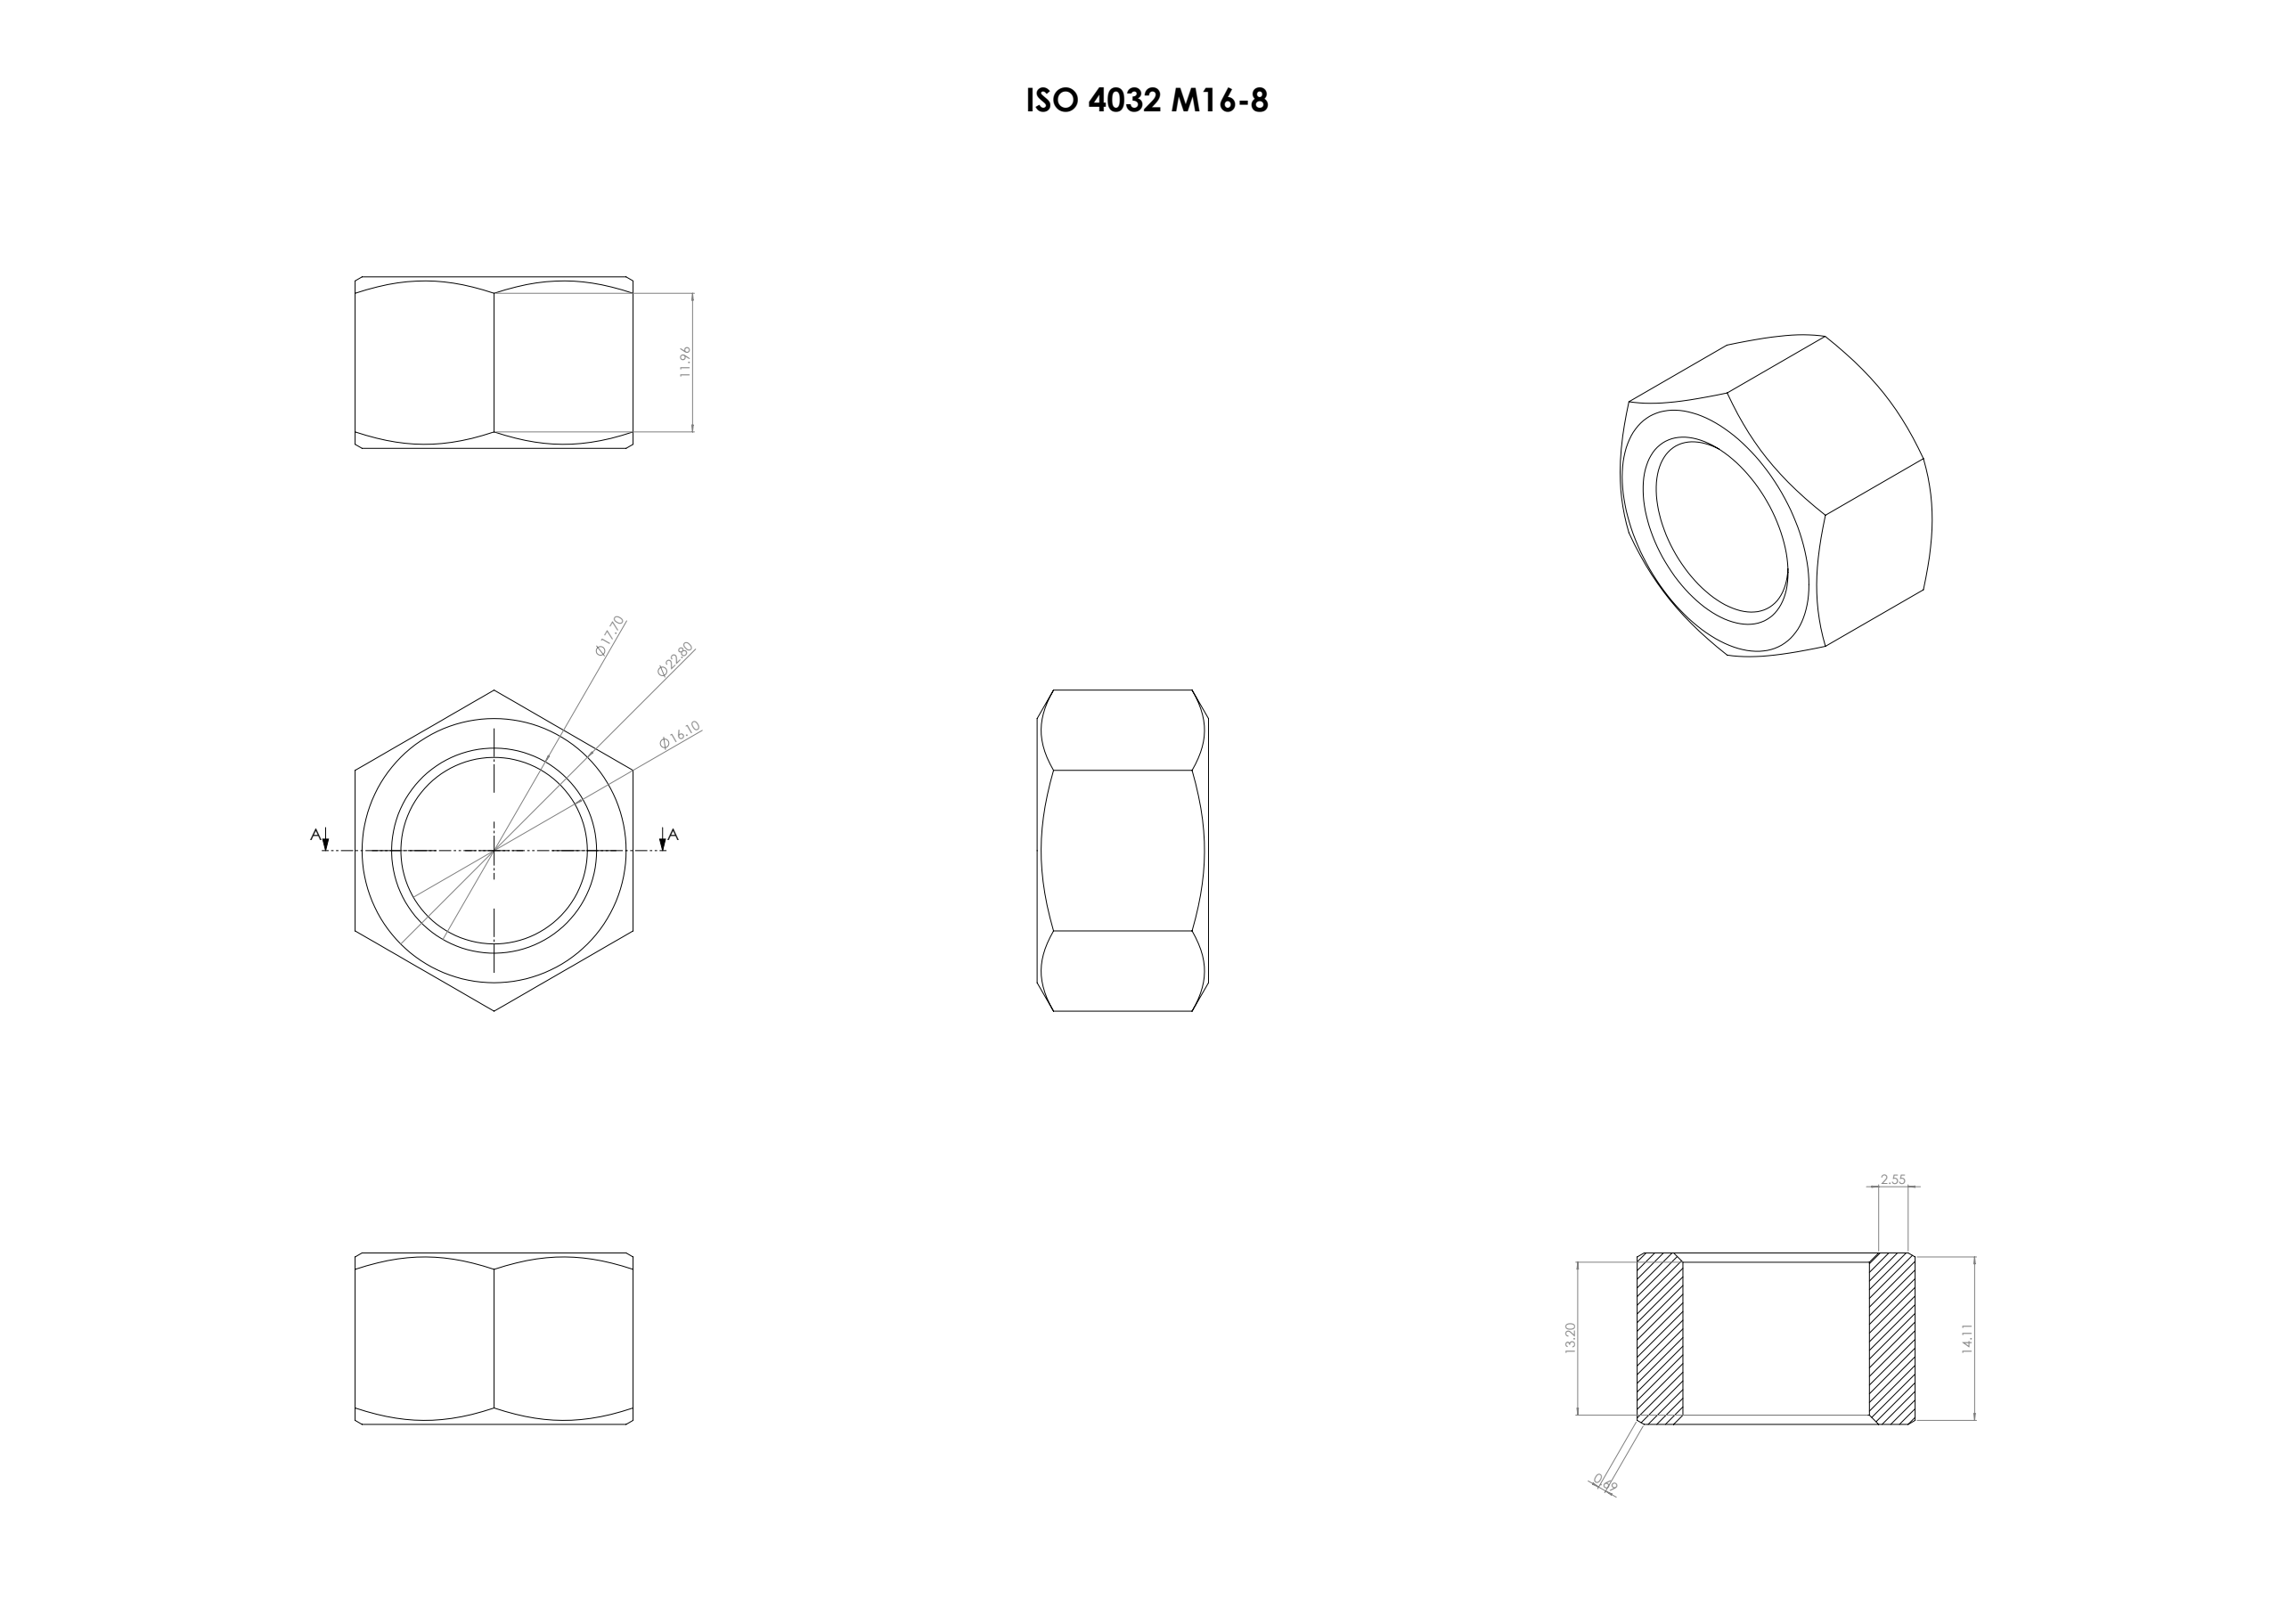
ISO-10303-21;
HEADER;
/* Generated by software containing ST-Developer
 * from STEP Tools, Inc. (www.steptools.com) 
 */

FILE_DESCRIPTION(
/* description */ (''),
/* implementation_level */ '2;1');

FILE_NAME(
/* name */ '18_ISO_4032_M16-8.step',
/* time_stamp */ '2026-10-20T10:03:03-07:00',
/* author */ (''),
/* organization */ (''),
/* preprocessor_version */ 'ST-DEVELOPER v20.2',
/* originating_system */ 'Autodesk Translation Framework v15.15.0.0',
/* authorisation */ '');

FILE_SCHEMA (('AUTOMOTIVE_DESIGN { 1 0 10303 214 3 1 1 }'));
ENDSEC;

DATA;
#10=MECHANICAL_DESIGN_GEOMETRIC_PRESENTATION_REPRESENTATION('',(#540),#71492);
#362=(
BOUNDED_CURVE()
B_SPLINE_CURVE(2,(#70596,#70597,#70598),.UNSPECIFIED.,.F.,.F.)
B_SPLINE_CURVE_WITH_KNOTS((3,3),(0.083069206448341,0.799733019594622),
 .UNSPECIFIED.)
CURVE()
GEOMETRIC_REPRESENTATION_ITEM()
RATIONAL_B_SPLINE_CURVE((1.01933756729741,1.09818360252296,1.09818360252296))
REPRESENTATION_ITEM('')
);
#363=(
BOUNDED_CURVE()
B_SPLINE_CURVE(2,(#70600,#70601,#70602),.UNSPECIFIED.,.F.,.F.)
B_SPLINE_CURVE_WITH_KNOTS((3,3),(0.0830692064483412,1.5163968327409),
 .UNSPECIFIED.)
CURVE()
GEOMETRIC_REPRESENTATION_ITEM()
RATIONAL_B_SPLINE_CURVE((1.01933756729741,1.17702963774851,1.01933756729741))
REPRESENTATION_ITEM('')
);
#364=(
BOUNDED_CURVE()
B_SPLINE_CURVE(2,(#70604,#70605,#70606),.UNSPECIFIED.,.F.,.F.)
B_SPLINE_CURVE_WITH_KNOTS((3,3),(0.0830692064483411,1.5163968327409),
 .UNSPECIFIED.)
CURVE()
GEOMETRIC_REPRESENTATION_ITEM()
RATIONAL_B_SPLINE_CURVE((1.01933756729741,1.17702963774851,1.01933756729741))
REPRESENTATION_ITEM('')
);
#365=(
BOUNDED_CURVE()
B_SPLINE_CURVE(2,(#70608,#70609,#70610),.UNSPECIFIED.,.F.,.F.)
B_SPLINE_CURVE_WITH_KNOTS((3,3),(0.0830692064483411,1.5163968327409),
 .UNSPECIFIED.)
CURVE()
GEOMETRIC_REPRESENTATION_ITEM()
RATIONAL_B_SPLINE_CURVE((1.01933756729741,1.17702963774851,1.01933756729741))
REPRESENTATION_ITEM('')
);
#366=(
BOUNDED_CURVE()
B_SPLINE_CURVE(2,(#70612,#70613,#70614),.UNSPECIFIED.,.F.,.F.)
B_SPLINE_CURVE_WITH_KNOTS((3,3),(0.083069206448341,1.5163968327409),
 .UNSPECIFIED.)
CURVE()
GEOMETRIC_REPRESENTATION_ITEM()
RATIONAL_B_SPLINE_CURVE((1.01933756729741,1.17702963774852,1.01933756729741))
REPRESENTATION_ITEM('')
);
#367=(
BOUNDED_CURVE()
B_SPLINE_CURVE(2,(#70616,#70617,#70618),.UNSPECIFIED.,.F.,.F.)
B_SPLINE_CURVE_WITH_KNOTS((3,3),(0.0830692064483414,1.5163968327409),
 .UNSPECIFIED.)
CURVE()
GEOMETRIC_REPRESENTATION_ITEM()
RATIONAL_B_SPLINE_CURVE((1.01933756729741,1.17702963774851,1.01933756729741))
REPRESENTATION_ITEM('')
);
#368=(
BOUNDED_CURVE()
B_SPLINE_CURVE(2,(#70619,#70620,#70621),.UNSPECIFIED.,.F.,.F.)
B_SPLINE_CURVE_WITH_KNOTS((3,3),(0.799733019594622,1.5163968327409),
 .UNSPECIFIED.)
CURVE()
GEOMETRIC_REPRESENTATION_ITEM()
RATIONAL_B_SPLINE_CURVE((1.09818360252296,1.09818360252296,1.01933756729741))
REPRESENTATION_ITEM('')
);
#369=(
BOUNDED_CURVE()
B_SPLINE_CURVE(2,(#70626,#70627,#70628),.UNSPECIFIED.,.F.,.F.)
B_SPLINE_CURVE_WITH_KNOTS((3,3),(0.0830692064483413,1.5163968327409),
 .UNSPECIFIED.)
CURVE()
GEOMETRIC_REPRESENTATION_ITEM()
RATIONAL_B_SPLINE_CURVE((1.01933756729741,1.17702963774851,1.01933756729741))
REPRESENTATION_ITEM('')
);
#370=(
BOUNDED_CURVE()
B_SPLINE_CURVE(2,(#70633,#70634,#70635),.UNSPECIFIED.,.F.,.F.)
B_SPLINE_CURVE_WITH_KNOTS((3,3),(0.0830692064483417,1.5163968327409),
 .UNSPECIFIED.)
CURVE()
GEOMETRIC_REPRESENTATION_ITEM()
RATIONAL_B_SPLINE_CURVE((1.01933756729741,1.17702963774851,1.01933756729741))
REPRESENTATION_ITEM('')
);
#371=(
BOUNDED_CURVE()
B_SPLINE_CURVE(2,(#70639,#70640,#70641),.UNSPECIFIED.,.F.,.F.)
B_SPLINE_CURVE_WITH_KNOTS((3,3),(0.0830692064483414,1.5163968327409),
 .UNSPECIFIED.)
CURVE()
GEOMETRIC_REPRESENTATION_ITEM()
RATIONAL_B_SPLINE_CURVE((1.01933756729741,1.17702963774851,1.01933756729741))
REPRESENTATION_ITEM('')
);
#372=(
BOUNDED_CURVE()
B_SPLINE_CURVE(2,(#70644,#70645,#70646),.UNSPECIFIED.,.F.,.F.)
B_SPLINE_CURVE_WITH_KNOTS((3,3),(0.0830692064483411,1.5163968327409),
 .UNSPECIFIED.)
CURVE()
GEOMETRIC_REPRESENTATION_ITEM()
RATIONAL_B_SPLINE_CURVE((1.01933756729741,1.17702963774851,1.01933756729741))
REPRESENTATION_ITEM('')
);
#373=(
BOUNDED_CURVE()
B_SPLINE_CURVE(2,(#70648,#70649,#70650),.UNSPECIFIED.,.F.,.F.)
B_SPLINE_CURVE_WITH_KNOTS((3,3),(0.799733019594622,1.5163968327409),
 .UNSPECIFIED.)
CURVE()
GEOMETRIC_REPRESENTATION_ITEM()
RATIONAL_B_SPLINE_CURVE((1.09818360252296,1.09818360252296,1.01933756729741))
REPRESENTATION_ITEM('')
);
#374=(
BOUNDED_CURVE()
B_SPLINE_CURVE(2,(#70653,#70654,#70655),.UNSPECIFIED.,.F.,.F.)
B_SPLINE_CURVE_WITH_KNOTS((3,3),(0.0830692064483414,0.799733019594622),
 .UNSPECIFIED.)
CURVE()
GEOMETRIC_REPRESENTATION_ITEM()
RATIONAL_B_SPLINE_CURVE((1.01933756729741,1.09818360252296,1.09818360252296))
REPRESENTATION_ITEM('')
);
#375=(
BOUNDED_CURVE()
B_SPLINE_CURVE(2,(#70656,#70657,#70658),.UNSPECIFIED.,.F.,.F.)
B_SPLINE_CURVE_WITH_KNOTS((3,3),(0.0830692064483413,1.5163968327409),
 .UNSPECIFIED.)
CURVE()
GEOMETRIC_REPRESENTATION_ITEM()
RATIONAL_B_SPLINE_CURVE((1.01933756729741,1.17702963774851,1.01933756729741))
REPRESENTATION_ITEM('')
);
#397=SHAPE_REPRESENTATION_RELATIONSHIP('SRR','None',#71618,#416);
#416=ADVANCED_BREP_SHAPE_REPRESENTATION('',(#435),#71488);
#435=MANIFOLD_SOLID_BREP('Nut',#28474);
#540=STYLED_ITEM('',(#71894),#435);
#1830=CYLINDRICAL_SURFACE('',#30448,0.805);
#1984=FACE_BOUND('',#6070,.T.);
#1985=FACE_BOUND('',#6073,.T.);
#2563=CIRCLE('',#30446,0.805);
#2564=CIRCLE('',#30447,0.885);
#2565=CIRCLE('',#30449,0.805);
#2566=CIRCLE('',#30451,1.14);
#2567=CIRCLE('',#30453,0.885);
#2568=CIRCLE('',#30455,1.14);
#2895=CONICAL_SURFACE('',#30445,0.845,0.785398163397448);
#2896=CONICAL_SURFACE('',#30452,0.845,0.785398163397448);
#2897=CONICAL_SURFACE('',#30456,1.28782032302755,1.0471975511966);
#2898=CONICAL_SURFACE('',#30460,1.28782032302755,1.0471975511966);
#4377=FACE_OUTER_BOUND('',#6067,.T.);
#4378=FACE_OUTER_BOUND('',#6068,.T.);
#4379=FACE_OUTER_BOUND('',#6069,.T.);
#4380=FACE_OUTER_BOUND('',#6071,.T.);
#4381=FACE_OUTER_BOUND('',#6072,.T.);
#4382=FACE_OUTER_BOUND('',#6074,.T.);
#4383=FACE_OUTER_BOUND('',#6075,.T.);
#4384=FACE_OUTER_BOUND('',#6076,.T.);
#4385=FACE_OUTER_BOUND('',#6077,.T.);
#4386=FACE_OUTER_BOUND('',#6078,.T.);
#4387=FACE_OUTER_BOUND('',#6079,.T.);
#4388=FACE_OUTER_BOUND('',#6080,.T.);
#4389=FACE_OUTER_BOUND('',#6081,.T.);
#6067=EDGE_LOOP('',(#25305,#25306,#25307,#25308));
#6068=EDGE_LOOP('',(#25309,#25310,#25311,#25312));
#6069=EDGE_LOOP('',(#25313));
#6070=EDGE_LOOP('',(#25314));
#6071=EDGE_LOOP('',(#25315,#25316,#25317,#25318));
#6072=EDGE_LOOP('',(#25319));
#6073=EDGE_LOOP('',(#25320));
#6074=EDGE_LOOP('',(#25321,#25322,#25323,#25324,#25325,#25326,#25327,#25328,
#25329,#25330));
#6075=EDGE_LOOP('',(#25331,#25332,#25333,#25334));
#6076=EDGE_LOOP('',(#25335,#25336,#25337,#25338));
#6077=EDGE_LOOP('',(#25339,#25340,#25341,#25342));
#6078=EDGE_LOOP('',(#25343,#25344,#25345,#25346,#25347,#25348,#25349,#25350,
#25351,#25352));
#6079=EDGE_LOOP('',(#25353,#25354,#25355,#25356));
#6080=EDGE_LOOP('',(#25357,#25358,#25359,#25360));
#6081=EDGE_LOOP('',(#25361,#25362,#25363,#25364,#25365,#25366));
#8589=LINE('',#70576,#11077);
#8590=LINE('',#70581,#11078);
#8591=LINE('',#70588,#11079);
#8592=LINE('',#70594,#11080);
#8593=LINE('',#70624,#11081);
#8594=LINE('',#70629,#11082);
#8595=LINE('',#70632,#11083);
#8596=LINE('',#70638,#11084);
#8597=LINE('',#70651,#11085);
#8598=LINE('',#70660,#11086);
#8599=LINE('',#70662,#11087);
#11077=VECTOR('',#36660,0.845);
#11078=VECTOR('',#36667,0.805);
#11079=VECTOR('',#36676,0.845);
#11080=VECTOR('',#36683,1.28782032302755);
#11081=VECTOR('',#36686,1.);
#11082=VECTOR('',#36687,1.);
#11083=VECTOR('',#36690,1.);
#11084=VECTOR('',#36693,1.);
#11085=VECTOR('',#36696,1.28782032302755);
#11086=VECTOR('',#36699,1.);
#11087=VECTOR('',#36702,1.);
#13617=VERTEX_POINT('',#70573);
#13618=VERTEX_POINT('',#70575);
#13619=VERTEX_POINT('',#70579);
#13620=VERTEX_POINT('',#70583);
#13621=VERTEX_POINT('',#70586);
#13622=VERTEX_POINT('',#70590);
#13623=VERTEX_POINT('',#70593);
#13624=VERTEX_POINT('',#70595);
#13625=VERTEX_POINT('',#70599);
#13626=VERTEX_POINT('',#70603);
#13627=VERTEX_POINT('',#70607);
#13628=VERTEX_POINT('',#70611);
#13629=VERTEX_POINT('',#70615);
#13630=VERTEX_POINT('',#70623);
#13631=VERTEX_POINT('',#70625);
#13632=VERTEX_POINT('',#70631);
#13633=VERTEX_POINT('',#70637);
#13634=VERTEX_POINT('',#70643);
#13635=VERTEX_POINT('',#70647);
#13636=VERTEX_POINT('',#70652);
#17536=EDGE_CURVE('',#13617,#13617,#2563,.T.);
#17537=EDGE_CURVE('',#13617,#13618,#8589,.T.);
#17538=EDGE_CURVE('',#13618,#13618,#2564,.T.);
#17539=EDGE_CURVE('',#13619,#13619,#2565,.T.);
#17540=EDGE_CURVE('',#13619,#13617,#8590,.T.);
#17541=EDGE_CURVE('',#13620,#13620,#2566,.T.);
#17542=EDGE_CURVE('',#13621,#13621,#2567,.T.);
#17543=EDGE_CURVE('',#13621,#13619,#8591,.T.);
#17544=EDGE_CURVE('',#13622,#13622,#2568,.T.);
#17545=EDGE_CURVE('',#13620,#13623,#8592,.T.);
#17546=EDGE_CURVE('',#13624,#13623,#362,.T.);
#17547=EDGE_CURVE('',#13625,#13624,#363,.T.);
#17548=EDGE_CURVE('',#13626,#13625,#364,.T.);
#17549=EDGE_CURVE('',#13627,#13626,#365,.T.);
#17550=EDGE_CURVE('',#13628,#13627,#366,.T.);
#17551=EDGE_CURVE('',#13629,#13628,#367,.T.);
#17552=EDGE_CURVE('',#13623,#13629,#368,.T.);
#17553=EDGE_CURVE('',#13627,#13630,#8593,.T.);
#17554=EDGE_CURVE('',#13630,#13631,#369,.T.);
#17555=EDGE_CURVE('',#13628,#13631,#8594,.T.);
#17556=EDGE_CURVE('',#13626,#13632,#8595,.T.);
#17557=EDGE_CURVE('',#13632,#13630,#370,.T.);
#17558=EDGE_CURVE('',#13625,#13633,#8596,.T.);
#17559=EDGE_CURVE('',#13633,#13632,#371,.T.);
#17560=EDGE_CURVE('',#13634,#13633,#372,.T.);
#17561=EDGE_CURVE('',#13635,#13634,#373,.T.);
#17562=EDGE_CURVE('',#13635,#13622,#8597,.T.);
#17563=EDGE_CURVE('',#13636,#13635,#374,.T.);
#17564=EDGE_CURVE('',#13631,#13636,#375,.T.);
#17565=EDGE_CURVE('',#13624,#13634,#8598,.T.);
#17566=EDGE_CURVE('',#13629,#13636,#8599,.T.);
#25305=ORIENTED_EDGE('',*,*,#17536,.T.);
#25306=ORIENTED_EDGE('',*,*,#17537,.T.);
#25307=ORIENTED_EDGE('',*,*,#17538,.T.);
#25308=ORIENTED_EDGE('',*,*,#17537,.F.);
#25309=ORIENTED_EDGE('',*,*,#17539,.F.);
#25310=ORIENTED_EDGE('',*,*,#17540,.T.);
#25311=ORIENTED_EDGE('',*,*,#17536,.F.);
#25312=ORIENTED_EDGE('',*,*,#17540,.F.);
#25313=ORIENTED_EDGE('',*,*,#17541,.T.);
#25314=ORIENTED_EDGE('',*,*,#17538,.F.);
#25315=ORIENTED_EDGE('',*,*,#17542,.T.);
#25316=ORIENTED_EDGE('',*,*,#17543,.T.);
#25317=ORIENTED_EDGE('',*,*,#17539,.T.);
#25318=ORIENTED_EDGE('',*,*,#17543,.F.);
#25319=ORIENTED_EDGE('',*,*,#17544,.T.);
#25320=ORIENTED_EDGE('',*,*,#17542,.F.);
#25321=ORIENTED_EDGE('',*,*,#17541,.F.);
#25322=ORIENTED_EDGE('',*,*,#17545,.T.);
#25323=ORIENTED_EDGE('',*,*,#17546,.F.);
#25324=ORIENTED_EDGE('',*,*,#17547,.F.);
#25325=ORIENTED_EDGE('',*,*,#17548,.F.);
#25326=ORIENTED_EDGE('',*,*,#17549,.F.);
#25327=ORIENTED_EDGE('',*,*,#17550,.F.);
#25328=ORIENTED_EDGE('',*,*,#17551,.F.);
#25329=ORIENTED_EDGE('',*,*,#17552,.F.);
#25330=ORIENTED_EDGE('',*,*,#17545,.F.);
#25331=ORIENTED_EDGE('',*,*,#17550,.T.);
#25332=ORIENTED_EDGE('',*,*,#17553,.T.);
#25333=ORIENTED_EDGE('',*,*,#17554,.T.);
#25334=ORIENTED_EDGE('',*,*,#17555,.F.);
#25335=ORIENTED_EDGE('',*,*,#17549,.T.);
#25336=ORIENTED_EDGE('',*,*,#17556,.T.);
#25337=ORIENTED_EDGE('',*,*,#17557,.T.);
#25338=ORIENTED_EDGE('',*,*,#17553,.F.);
#25339=ORIENTED_EDGE('',*,*,#17548,.T.);
#25340=ORIENTED_EDGE('',*,*,#17558,.T.);
#25341=ORIENTED_EDGE('',*,*,#17559,.T.);
#25342=ORIENTED_EDGE('',*,*,#17556,.F.);
#25343=ORIENTED_EDGE('',*,*,#17554,.F.);
#25344=ORIENTED_EDGE('',*,*,#17557,.F.);
#25345=ORIENTED_EDGE('',*,*,#17559,.F.);
#25346=ORIENTED_EDGE('',*,*,#17560,.F.);
#25347=ORIENTED_EDGE('',*,*,#17561,.F.);
#25348=ORIENTED_EDGE('',*,*,#17562,.T.);
#25349=ORIENTED_EDGE('',*,*,#17544,.F.);
#25350=ORIENTED_EDGE('',*,*,#17562,.F.);
#25351=ORIENTED_EDGE('',*,*,#17563,.F.);
#25352=ORIENTED_EDGE('',*,*,#17564,.F.);
#25353=ORIENTED_EDGE('',*,*,#17547,.T.);
#25354=ORIENTED_EDGE('',*,*,#17565,.T.);
#25355=ORIENTED_EDGE('',*,*,#17560,.T.);
#25356=ORIENTED_EDGE('',*,*,#17558,.F.);
#25357=ORIENTED_EDGE('',*,*,#17551,.T.);
#25358=ORIENTED_EDGE('',*,*,#17555,.T.);
#25359=ORIENTED_EDGE('',*,*,#17564,.T.);
#25360=ORIENTED_EDGE('',*,*,#17566,.F.);
#25361=ORIENTED_EDGE('',*,*,#17546,.T.);
#25362=ORIENTED_EDGE('',*,*,#17552,.T.);
#25363=ORIENTED_EDGE('',*,*,#17566,.T.);
#25364=ORIENTED_EDGE('',*,*,#17563,.T.);
#25365=ORIENTED_EDGE('',*,*,#17561,.T.);
#25366=ORIENTED_EDGE('',*,*,#17565,.F.);
#26825=PLANE('',#30450);
#26826=PLANE('',#30454);
#26827=PLANE('',#30457);
#26828=PLANE('',#30458);
#26829=PLANE('',#30459);
#26830=PLANE('',#30461);
#26831=PLANE('',#30462);
#26832=PLANE('',#30463);
#28285=ADVANCED_FACE('',(#4377),#2895,.F.);
#28286=ADVANCED_FACE('',(#4378),#1830,.F.);
#28287=ADVANCED_FACE('',(#4379,#1984),#26825,.F.);
#28288=ADVANCED_FACE('',(#4380),#2896,.F.);
#28289=ADVANCED_FACE('',(#4381,#1985),#26826,.T.);
#28290=ADVANCED_FACE('',(#4382),#2897,.T.);
#28291=ADVANCED_FACE('',(#4383),#26827,.T.);
#28292=ADVANCED_FACE('',(#4384),#26828,.T.);
#28293=ADVANCED_FACE('',(#4385),#26829,.T.);
#28294=ADVANCED_FACE('',(#4386),#2898,.T.);
#28295=ADVANCED_FACE('',(#4387),#26830,.T.);
#28296=ADVANCED_FACE('',(#4388),#26831,.T.);
#28297=ADVANCED_FACE('',(#4389),#26832,.T.);
#28474=CLOSED_SHELL('',(#28285,#28286,#28287,#28288,#28289,#28290,#28291,
#28292,#28293,#28294,#28295,#28296,#28297));
#30444=AXIS2_PLACEMENT_3D('',#70571,#36654,#36655);
#30445=AXIS2_PLACEMENT_3D('',#70572,#36656,#36657);
#30446=AXIS2_PLACEMENT_3D('',#70574,#36658,#36659);
#30447=AXIS2_PLACEMENT_3D('',#70577,#36661,#36662);
#30448=AXIS2_PLACEMENT_3D('',#70578,#36663,#36664);
#30449=AXIS2_PLACEMENT_3D('',#70580,#36665,#36666);
#30450=AXIS2_PLACEMENT_3D('',#70582,#36668,#36669);
#30451=AXIS2_PLACEMENT_3D('',#70584,#36670,#36671);
#30452=AXIS2_PLACEMENT_3D('',#70585,#36672,#36673);
#30453=AXIS2_PLACEMENT_3D('',#70587,#36674,#36675);
#30454=AXIS2_PLACEMENT_3D('',#70589,#36677,#36678);
#30455=AXIS2_PLACEMENT_3D('',#70591,#36679,#36680);
#30456=AXIS2_PLACEMENT_3D('',#70592,#36681,#36682);
#30457=AXIS2_PLACEMENT_3D('',#70622,#36684,#36685);
#30458=AXIS2_PLACEMENT_3D('',#70630,#36688,#36689);
#30459=AXIS2_PLACEMENT_3D('',#70636,#36691,#36692);
#30460=AXIS2_PLACEMENT_3D('',#70642,#36694,#36695);
#30461=AXIS2_PLACEMENT_3D('',#70659,#36697,#36698);
#30462=AXIS2_PLACEMENT_3D('',#70661,#36700,#36701);
#30463=AXIS2_PLACEMENT_3D('',#70663,#36703,#36704);
#36654=DIRECTION('axis',(0.,0.,1.));
#36655=DIRECTION('refdir',(1.,0.,0.));
#36656=DIRECTION('center_axis',(0.,0.,-1.));
#36657=DIRECTION('ref_axis',(1.,0.,0.));
#36658=DIRECTION('center_axis',(0.,0.,1.));
#36659=DIRECTION('ref_axis',(1.,0.,0.));
#36660=DIRECTION('',(-0.707106781186547,-8.65956056235493E-17,-0.707106781186548));
#36661=DIRECTION('center_axis',(0.,0.,-1.));
#36662=DIRECTION('ref_axis',(1.,0.,0.));
#36663=DIRECTION('center_axis',(0.,0.,1.));
#36664=DIRECTION('ref_axis',(1.,0.,0.));
#36665=DIRECTION('center_axis',(0.,0.,-1.));
#36666=DIRECTION('ref_axis',(1.,0.,0.));
#36667=DIRECTION('',(0.,0.,-1.));
#36668=DIRECTION('center_axis',(0.,0.,1.));
#36669=DIRECTION('ref_axis',(1.,0.,0.));
#36670=DIRECTION('center_axis',(0.,0.,-1.));
#36671=DIRECTION('ref_axis',(1.,0.,0.));
#36672=DIRECTION('center_axis',(0.,0.,1.));
#36673=DIRECTION('ref_axis',(1.,0.,0.));
#36674=DIRECTION('center_axis',(0.,0.,1.));
#36675=DIRECTION('ref_axis',(1.,0.,0.));
#36676=DIRECTION('',(0.707106781186547,8.65956056235493E-17,-0.707106781186548));
#36677=DIRECTION('center_axis',(0.,0.,1.));
#36678=DIRECTION('ref_axis',(1.,0.,0.));
#36679=DIRECTION('center_axis',(0.,0.,1.));
#36680=DIRECTION('ref_axis',(1.,0.,0.));
#36681=DIRECTION('center_axis',(0.,0.,1.));
#36682=DIRECTION('ref_axis',(1.,0.,0.));
#36683=DIRECTION('',(-0.866025403784439,-1.06057523872491E-16,0.5));
#36684=DIRECTION('center_axis',(0.5,-0.866025403784439,0.));
#36685=DIRECTION('ref_axis',(0.866025403784439,0.5,0.));
#36686=DIRECTION('',(0.,0.,1.));
#36687=DIRECTION('',(0.,0.,1.));
#36688=DIRECTION('center_axis',(1.,-3.20493781063927E-16,0.));
#36689=DIRECTION('ref_axis',(3.20493781063927E-16,1.,0.));
#36690=DIRECTION('',(0.,0.,1.));
#36691=DIRECTION('center_axis',(0.5,0.866025403784439,0.));
#36692=DIRECTION('ref_axis',(-0.866025403784439,0.5,0.));
#36693=DIRECTION('',(0.,0.,1.));
#36694=DIRECTION('center_axis',(0.,0.,-1.));
#36695=DIRECTION('ref_axis',(1.,0.,0.));
#36696=DIRECTION('',(0.866025403784439,1.06057523872491E-16,0.5));
#36697=DIRECTION('center_axis',(-0.5,0.866025403784439,0.));
#36698=DIRECTION('ref_axis',(-0.866025403784439,-0.5,0.));
#36699=DIRECTION('',(0.,0.,1.));
#36700=DIRECTION('center_axis',(-0.5,-0.866025403784439,0.));
#36701=DIRECTION('ref_axis',(0.866025403784439,-0.5,0.));
#36702=DIRECTION('',(0.,0.,1.));
#36703=DIRECTION('center_axis',(-1.,-1.60246890531964E-16,0.));
#36704=DIRECTION('ref_axis',(1.60246890531964E-16,-1.,0.));
#70571=CARTESIAN_POINT('',(0.,0.,0.));
#70572=CARTESIAN_POINT('Origin',(0.,0.,0.04));
#70573=CARTESIAN_POINT('',(-0.805,-9.85840673313619E-17,0.08));
#70574=CARTESIAN_POINT('Origin',(0.,0.,0.08));
#70575=CARTESIAN_POINT('',(-0.885,1.08381241724541E-16,0.));
#70576=CARTESIAN_POINT('',(-0.845,-1.03482654527951E-16,0.04));
#70577=CARTESIAN_POINT('Origin',(0.,0.,0.));
#70578=CARTESIAN_POINT('Origin',(0.,0.,0.));
#70579=CARTESIAN_POINT('',(-0.805,9.85840673313619E-17,1.4));
#70580=CARTESIAN_POINT('Origin',(0.,0.,1.4));
#70581=CARTESIAN_POINT('',(-0.805,-9.85840673313619E-17,0.));
#70582=CARTESIAN_POINT('Origin',(0.,0.,0.));
#70583=CARTESIAN_POINT('',(-1.14,-1.39609735102798E-16,-8.32667268468867E-17));
#70584=CARTESIAN_POINT('Origin',(0.,0.,0.));
#70585=CARTESIAN_POINT('Origin',(0.,0.,1.44));
#70586=CARTESIAN_POINT('',(-0.885,-1.08381241724541E-16,1.48));
#70587=CARTESIAN_POINT('Origin',(0.,0.,1.48));
#70588=CARTESIAN_POINT('',(-0.845,-1.03482654527951E-16,1.44));
#70589=CARTESIAN_POINT('Origin',(0.,0.,1.48));
#70590=CARTESIAN_POINT('',(-1.14,-1.39609735102798E-16,1.48));
#70591=CARTESIAN_POINT('Origin',(0.,0.,1.48));
#70592=CARTESIAN_POINT('Origin',(0.,0.,0.085344103291654));
#70593=CARTESIAN_POINT('',(-1.2,-1.36663997456004E-16,0.0346410161513778));
#70594=CARTESIAN_POINT('',(-1.28782032302755,-1.5771250364726E-16,0.085344103291654));
#70595=CARTESIAN_POINT('',(-1.2,0.692820323027551,0.141820693123827));
#70596=CARTESIAN_POINT('Ctrl Pts',(-1.2,0.692820323027551,0.141820693123827));
#70597=CARTESIAN_POINT('Ctrl Pts',(-1.2,0.321539030917347,0.0346410161513777));
#70598=CARTESIAN_POINT('Ctrl Pts',(-1.2,-1.26370379014326E-16,0.0346410161513778));
#70599=CARTESIAN_POINT('',(8.48460190979925E-17,1.3856406460551,0.141820693123827));
#70600=CARTESIAN_POINT('Ctrl Pts',(8.48460190979925E-17,1.3856406460551,
0.141820693123827));
#70601=CARTESIAN_POINT('Ctrl Pts',(-0.599999999999999,1.03923048454133,
-0.0581793068761738));
#70602=CARTESIAN_POINT('Ctrl Pts',(-1.2,0.692820323027551,0.141820693123827));
#70603=CARTESIAN_POINT('',(1.2,0.692820323027551,0.141820693123827));
#70604=CARTESIAN_POINT('Ctrl Pts',(1.2,0.692820323027551,0.141820693123827));
#70605=CARTESIAN_POINT('Ctrl Pts',(0.6,1.03923048454133,-0.0581793068761734));
#70606=CARTESIAN_POINT('Ctrl Pts',(8.48460190979925E-17,1.3856406460551,
0.141820693123827));
#70607=CARTESIAN_POINT('',(1.2,-0.692820323027552,0.141820693123827));
#70608=CARTESIAN_POINT('Ctrl Pts',(1.2,-0.692820323027552,0.141820693123827));
#70609=CARTESIAN_POINT('Ctrl Pts',(1.2,-9.99200722162641E-16,-0.0581793068761738));
#70610=CARTESIAN_POINT('Ctrl Pts',(1.2,0.692820323027551,0.141820693123827));
#70611=CARTESIAN_POINT('',(-2.54538057293978E-16,-1.3856406460551,0.141820693123827));
#70612=CARTESIAN_POINT('Ctrl Pts',(-2.54538057293978E-16,-1.3856406460551,
0.141820693123827));
#70613=CARTESIAN_POINT('Ctrl Pts',(0.6,-1.03923048454133,-0.0581793068761735));
#70614=CARTESIAN_POINT('Ctrl Pts',(1.2,-0.692820323027551,0.141820693123827));
#70615=CARTESIAN_POINT('',(-1.2,-0.692820323027551,0.141820693123827));
#70616=CARTESIAN_POINT('Ctrl Pts',(-1.2,-0.692820323027551,0.141820693123827));
#70617=CARTESIAN_POINT('Ctrl Pts',(-0.6,-1.03923048454133,-0.0581793068761732));
#70618=CARTESIAN_POINT('Ctrl Pts',(-2.54538057293978E-16,-1.3856406460551,
0.141820693123827));
#70619=CARTESIAN_POINT('Ctrl Pts',(-1.2,-1.26370379014326E-16,0.0346410161513778));
#70620=CARTESIAN_POINT('Ctrl Pts',(-1.2,-0.321539030917348,0.0346410161513778));
#70621=CARTESIAN_POINT('Ctrl Pts',(-1.2,-0.692820323027551,0.141820693123827));
#70622=CARTESIAN_POINT('Origin',(-2.54538057293978E-16,-1.3856406460551,
0.));
#70623=CARTESIAN_POINT('',(1.2,-0.692820323027552,1.33817930687617));
#70624=CARTESIAN_POINT('',(1.2,-0.692820323027552,0.));
#70625=CARTESIAN_POINT('',(-2.54538057293978E-16,-1.3856406460551,1.33817930687617));
#70626=CARTESIAN_POINT('Ctrl Pts',(1.2,-0.692820323027552,1.33817930687617));
#70627=CARTESIAN_POINT('Ctrl Pts',(0.6,-1.03923048454133,1.53817930687617));
#70628=CARTESIAN_POINT('Ctrl Pts',(-2.54538057293978E-16,-1.3856406460551,
1.33817930687617));
#70629=CARTESIAN_POINT('',(-2.54538057293978E-16,-1.3856406460551,0.));
#70630=CARTESIAN_POINT('Origin',(1.2,-0.692820323027552,0.));
#70631=CARTESIAN_POINT('',(1.2,0.692820323027551,1.33817930687617));
#70632=CARTESIAN_POINT('',(1.2,0.692820323027551,0.));
#70633=CARTESIAN_POINT('Ctrl Pts',(1.2,0.692820323027551,1.33817930687617));
#70634=CARTESIAN_POINT('Ctrl Pts',(1.2,0.,1.53817930687617));
#70635=CARTESIAN_POINT('Ctrl Pts',(1.2,-0.692820323027552,1.33817930687617));
#70636=CARTESIAN_POINT('Origin',(1.2,0.692820323027551,0.));
#70637=CARTESIAN_POINT('',(8.48460190979925E-17,1.3856406460551,1.33817930687617));
#70638=CARTESIAN_POINT('',(8.48460190979926E-17,1.3856406460551,0.));
#70639=CARTESIAN_POINT('Ctrl Pts',(8.48460190979925E-17,1.3856406460551,
1.33817930687617));
#70640=CARTESIAN_POINT('Ctrl Pts',(0.6,1.03923048454133,1.53817930687617));
#70641=CARTESIAN_POINT('Ctrl Pts',(1.2,0.692820323027551,1.33817930687617));
#70642=CARTESIAN_POINT('Origin',(0.,0.,1.39465589670835));
#70643=CARTESIAN_POINT('',(-1.2,0.692820323027551,1.33817930687617));
#70644=CARTESIAN_POINT('Ctrl Pts',(-1.2,0.692820323027551,1.33817930687617));
#70645=CARTESIAN_POINT('Ctrl Pts',(-0.6,1.03923048454133,1.53817930687617));
#70646=CARTESIAN_POINT('Ctrl Pts',(8.48460190979925E-17,1.3856406460551,
1.33817930687617));
#70647=CARTESIAN_POINT('',(-1.2,-1.36663997456004E-16,1.44535898384862));
#70648=CARTESIAN_POINT('Ctrl Pts',(-1.2,-1.26370379014326E-16,1.44535898384862));
#70649=CARTESIAN_POINT('Ctrl Pts',(-1.2,0.321539030917347,1.44535898384862));
#70650=CARTESIAN_POINT('Ctrl Pts',(-1.2,0.692820323027551,1.33817930687617));
#70651=CARTESIAN_POINT('',(-1.28782032302755,-1.5771250364726E-16,1.39465589670835));
#70652=CARTESIAN_POINT('',(-1.2,-0.692820323027551,1.33817930687617));
#70653=CARTESIAN_POINT('Ctrl Pts',(-1.2,-0.692820323027551,1.33817930687617));
#70654=CARTESIAN_POINT('Ctrl Pts',(-1.2,-0.321539030917348,1.44535898384862));
#70655=CARTESIAN_POINT('Ctrl Pts',(-1.2,-1.26370379014326E-16,1.44535898384862));
#70656=CARTESIAN_POINT('Ctrl Pts',(-2.54538057293978E-16,-1.3856406460551,
1.33817930687617));
#70657=CARTESIAN_POINT('Ctrl Pts',(-0.6,-1.03923048454133,1.53817930687617));
#70658=CARTESIAN_POINT('Ctrl Pts',(-1.2,-0.692820323027551,1.33817930687617));
#70659=CARTESIAN_POINT('Origin',(8.48460190979926E-17,1.3856406460551,0.));
#70660=CARTESIAN_POINT('',(-1.2,0.692820323027551,0.));
#70661=CARTESIAN_POINT('Origin',(-1.2,-0.692820323027551,0.));
#70662=CARTESIAN_POINT('',(-1.2,-0.692820323027551,0.));
#70663=CARTESIAN_POINT('Origin',(-1.2,0.692820323027551,0.));
#71467=UNCERTAINTY_MEASURE_WITH_UNIT(LENGTH_MEASURE(0.001),#71493,
'DISTANCE_ACCURACY_VALUE',
'Maximum model space distance between geometric entities at asserted c
onnectivities');
#71471=UNCERTAINTY_MEASURE_WITH_UNIT(LENGTH_MEASURE(0.001),#71493,
'DISTANCE_ACCURACY_VALUE',
'Maximum model space distance between geometric entities at asserted c
onnectivities');
#71488=(
GEOMETRIC_REPRESENTATION_CONTEXT(3)
GLOBAL_UNCERTAINTY_ASSIGNED_CONTEXT((#71467))
GLOBAL_UNIT_ASSIGNED_CONTEXT((#71493,#71495,#71496))
REPRESENTATION_CONTEXT('','3D')
);
#71492=(
GEOMETRIC_REPRESENTATION_CONTEXT(3)
GLOBAL_UNCERTAINTY_ASSIGNED_CONTEXT((#71471))
GLOBAL_UNIT_ASSIGNED_CONTEXT((#71493,#71495,#71496))
REPRESENTATION_CONTEXT('','3D')
);
#71493=(
LENGTH_UNIT()
NAMED_UNIT(*)
SI_UNIT(.CENTI.,.METRE.)
);
#71495=(
NAMED_UNIT(*)
PLANE_ANGLE_UNIT()
SI_UNIT($,.RADIAN.)
);
#71496=(
NAMED_UNIT(*)
SI_UNIT($,.STERADIAN.)
SOLID_ANGLE_UNIT()
);
#71513=SHAPE_DEFINITION_REPRESENTATION(#71533,#71618);
#71533=PRODUCT_DEFINITION_SHAPE('',$,#71639);
#71618=SHAPE_REPRESENTATION('',(#30444),#71488);
#71622=PRODUCT_DEFINITION_CONTEXT('part definition',#71684,'design');
#71639=PRODUCT_DEFINITION('2026-10-19-03-23-16-216','18_ISO_4032_M16-8',
#71659,#71622);
#71659=PRODUCT_DEFINITION_FORMATION('',$,#71702);
#71684=APPLICATION_CONTEXT(
'Core Data for Automotive Mechanical Design Process');
#71685=PRODUCT_CONTEXT('part definition',#71684,'mechanical');
#71702=PRODUCT('2026-10-19-03-23-16-216','18_ISO_4032_M16-8',$,(#71685));
#71888=COLOUR_RGB('Black',0.12,0.14,0.17);
#71889=FILL_AREA_STYLE_COLOUR('',#71888);
#71890=FILL_AREA_STYLE('',(#71889));
#71891=SURFACE_STYLE_FILL_AREA(#71890);
#71892=SURFACE_SIDE_STYLE('',(#71891));
#71893=SURFACE_STYLE_USAGE(.BOTH.,#71892);
#71894=PRESENTATION_STYLE_ASSIGNMENT((#71893));
ENDSEC;
END-ISO-10303-21;
